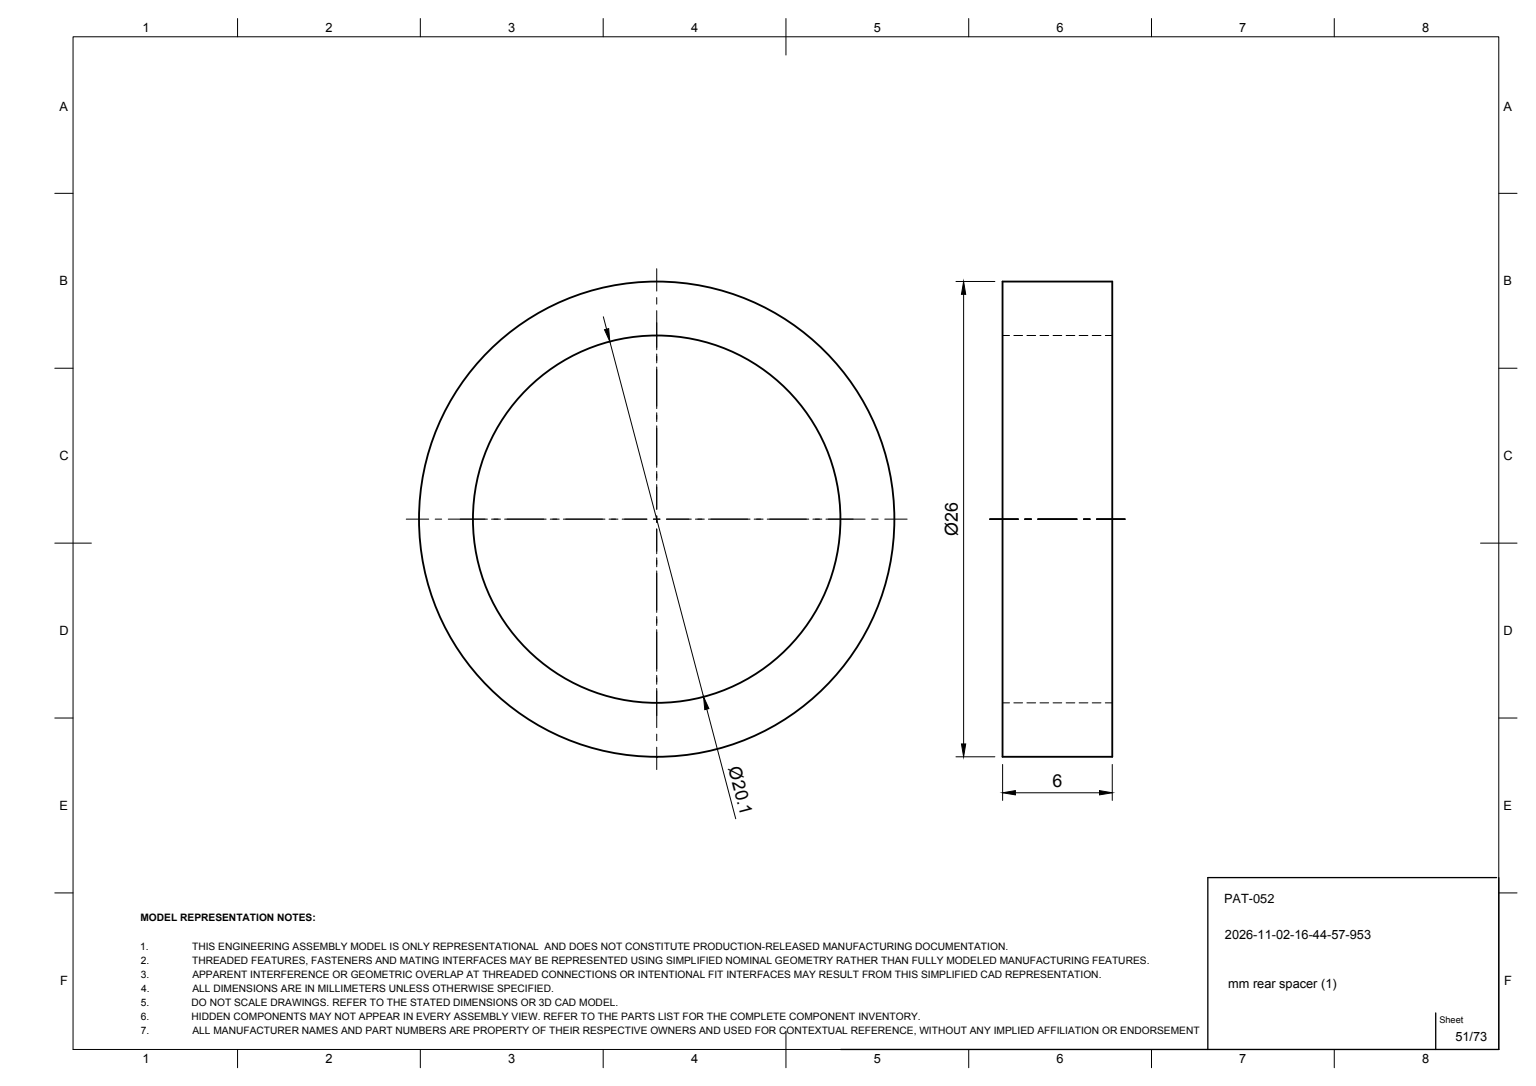
ISO-10303-21;
HEADER;
/* Generated by software containing ST-Developer
 * from STEP Tools, Inc. (www.steptools.com) 
 */

FILE_DESCRIPTION(
/* description */ ('Hand-crank gear train demonstrator'),
/* implementation_level */ '2;1');

FILE_NAME(
/* name */ 'mm rear spacer (1).step',
/* time_stamp */ '2026-10-28T03:22:13-07:00',
/* author */ (''),
/* organization */ (''),
/* preprocessor_version */ 'ST-DEVELOPER v20.2',
/* originating_system */ 'Autodesk Translation Framework v15.17.0.0',
/* authorisation */ '');

FILE_SCHEMA (('AUTOMOTIVE_DESIGN { 1 0 10303 214 3 1 1 }'));
ENDSEC;

DATA;
#10=MECHANICAL_DESIGN_GEOMETRIC_PRESENTATION_REPRESENTATION('',(#1245),#62758);
#1102=SHAPE_REPRESENTATION_RELATIONSHIP('SRR','None',#63078,#1166);
#1166=ADVANCED_BREP_SHAPE_REPRESENTATION('',(#1320),#62732);
#1245=STYLED_ITEM('',(#63476),#1320);
#1320=MANIFOLD_SOLID_BREP('Body1',#16429);
#1578=FACE_BOUND('',#3825,.T.);
#1579=FACE_BOUND('',#3827,.T.);
#1949=PLANE('',#18177);
#1950=PLANE('',#18178);
#2650=FACE_OUTER_BOUND('',#3822,.T.);
#2651=FACE_OUTER_BOUND('',#3823,.T.);
#2652=FACE_OUTER_BOUND('',#3824,.T.);
#2653=FACE_OUTER_BOUND('',#3826,.T.);
#3822=EDGE_LOOP('',(#13083,#13084,#13085,#13086));
#3823=EDGE_LOOP('',(#13087,#13088,#13089,#13090));
#3824=EDGE_LOOP('',(#13091));
#3825=EDGE_LOOP('',(#13092));
#3826=EDGE_LOOP('',(#13093));
#3827=EDGE_LOOP('',(#13094));
#4946=LINE('',#26469,#6078);
#4947=LINE('',#26475,#6079);
#6078=VECTOR('',#21521,1.005);
#6079=VECTOR('',#21528,1.3);
#6978=CIRCLE('',#18172,1.005);
#6979=CIRCLE('',#18173,1.005);
#6980=CIRCLE('',#18175,1.3);
#6981=CIRCLE('',#18176,1.3);
#7975=VERTEX_POINT('',#26466);
#7976=VERTEX_POINT('',#26468);
#7977=VERTEX_POINT('',#26472);
#7978=VERTEX_POINT('',#26474);
#9793=EDGE_CURVE('',#7975,#7975,#6978,.T.);
#9794=EDGE_CURVE('',#7975,#7976,#4946,.T.);
#9795=EDGE_CURVE('',#7976,#7976,#6979,.T.);
#9796=EDGE_CURVE('',#7977,#7977,#6980,.T.);
#9797=EDGE_CURVE('',#7977,#7978,#4947,.T.);
#9798=EDGE_CURVE('',#7978,#7978,#6981,.T.);
#13083=ORIENTED_EDGE('',*,*,#9793,.F.);
#13084=ORIENTED_EDGE('',*,*,#9794,.T.);
#13085=ORIENTED_EDGE('',*,*,#9795,.T.);
#13086=ORIENTED_EDGE('',*,*,#9794,.F.);
#13087=ORIENTED_EDGE('',*,*,#9796,.F.);
#13088=ORIENTED_EDGE('',*,*,#9797,.T.);
#13089=ORIENTED_EDGE('',*,*,#9798,.T.);
#13090=ORIENTED_EDGE('',*,*,#9797,.F.);
#13091=ORIENTED_EDGE('',*,*,#9796,.T.);
#13092=ORIENTED_EDGE('',*,*,#9793,.T.);
#13093=ORIENTED_EDGE('',*,*,#9798,.F.);
#13094=ORIENTED_EDGE('',*,*,#9795,.F.);
#15324=CYLINDRICAL_SURFACE('',#18171,1.005);
#15325=CYLINDRICAL_SURFACE('',#18174,1.3);
#15960=ADVANCED_FACE('',(#2650),#15324,.F.);
#15961=ADVANCED_FACE('',(#2651),#15325,.T.);
#15962=ADVANCED_FACE('',(#2652,#1578),#1949,.T.);
#15963=ADVANCED_FACE('',(#2653,#1579),#1950,.F.);
#16429=CLOSED_SHELL('',(#15960,#15961,#15962,#15963));
#18170=AXIS2_PLACEMENT_3D('',#26464,#21515,#21516);
#18171=AXIS2_PLACEMENT_3D('',#26465,#21517,#21518);
#18172=AXIS2_PLACEMENT_3D('',#26467,#21519,#21520);
#18173=AXIS2_PLACEMENT_3D('',#26470,#21522,#21523);
#18174=AXIS2_PLACEMENT_3D('',#26471,#21524,#21525);
#18175=AXIS2_PLACEMENT_3D('',#26473,#21526,#21527);
#18176=AXIS2_PLACEMENT_3D('',#26476,#21529,#21530);
#18177=AXIS2_PLACEMENT_3D('',#26477,#21531,#21532);
#18178=AXIS2_PLACEMENT_3D('',#26478,#21533,#21534);
#21515=DIRECTION('axis',(0.,0.,1.));
#21516=DIRECTION('refdir',(1.,0.,0.));
#21517=DIRECTION('center_axis',(0.,1.,0.));
#21518=DIRECTION('ref_axis',(1.,0.,0.));
#21519=DIRECTION('center_axis',(0.,-1.,0.));
#21520=DIRECTION('ref_axis',(1.,0.,0.));
#21521=DIRECTION('',(0.,-1.,0.));
#21522=DIRECTION('center_axis',(0.,-1.,0.));
#21523=DIRECTION('ref_axis',(1.,0.,0.));
#21524=DIRECTION('center_axis',(0.,1.,0.));
#21525=DIRECTION('ref_axis',(1.,0.,0.));
#21526=DIRECTION('center_axis',(0.,1.,0.));
#21527=DIRECTION('ref_axis',(1.,0.,0.));
#21528=DIRECTION('',(0.,-1.,0.));
#21529=DIRECTION('center_axis',(0.,1.,0.));
#21530=DIRECTION('ref_axis',(1.,0.,0.));
#21531=DIRECTION('center_axis',(0.,1.,0.));
#21532=DIRECTION('ref_axis',(1.,0.,0.));
#21533=DIRECTION('center_axis',(0.,1.,0.));
#21534=DIRECTION('ref_axis',(1.,0.,0.));
#26464=CARTESIAN_POINT('',(0.,0.,0.));
#26465=CARTESIAN_POINT('Origin',(6.,-2.8,9.));
#26466=CARTESIAN_POINT('',(4.995,-2.2,9.));
#26467=CARTESIAN_POINT('Origin',(6.,-2.2,9.));
#26468=CARTESIAN_POINT('',(4.995,-2.8,9.));
#26469=CARTESIAN_POINT('',(4.995,-2.8,9.));
#26470=CARTESIAN_POINT('Origin',(6.,-2.8,9.));
#26471=CARTESIAN_POINT('Origin',(6.,-2.8,9.));
#26472=CARTESIAN_POINT('',(4.7,-2.2,9.));
#26473=CARTESIAN_POINT('Origin',(6.,-2.2,9.));
#26474=CARTESIAN_POINT('',(4.7,-2.8,9.));
#26475=CARTESIAN_POINT('',(4.7,-2.8,9.));
#26476=CARTESIAN_POINT('Origin',(6.,-2.8,9.));
#26477=CARTESIAN_POINT('Origin',(6.,-2.2,9.));
#26478=CARTESIAN_POINT('Origin',(6.,-2.8,9.));
#62658=UNCERTAINTY_MEASURE_WITH_UNIT(LENGTH_MEASURE(0.001),#62759,
'DISTANCE_ACCURACY_VALUE',
'Maximum model space distance between geometric entities at asserted c
onnectivities');
#62684=UNCERTAINTY_MEASURE_WITH_UNIT(LENGTH_MEASURE(0.001),#62759,
'DISTANCE_ACCURACY_VALUE',
'Maximum model space distance between geometric entities at asserted c
onnectivities');
#62732=(
GEOMETRIC_REPRESENTATION_CONTEXT(3)
GLOBAL_UNCERTAINTY_ASSIGNED_CONTEXT((#62658))
GLOBAL_UNIT_ASSIGNED_CONTEXT((#62759,#62761,#62762))
REPRESENTATION_CONTEXT('','3D')
);
#62758=(
GEOMETRIC_REPRESENTATION_CONTEXT(3)
GLOBAL_UNCERTAINTY_ASSIGNED_CONTEXT((#62684))
GLOBAL_UNIT_ASSIGNED_CONTEXT((#62759,#62761,#62762))
REPRESENTATION_CONTEXT('','3D')
);
#62759=(
LENGTH_UNIT()
NAMED_UNIT(*)
SI_UNIT(.CENTI.,.METRE.)
);
#62761=(
NAMED_UNIT(*)
PLANE_ANGLE_UNIT()
SI_UNIT($,.RADIAN.)
);
#62762=(
NAMED_UNIT(*)
SI_UNIT($,.STERADIAN.)
SOLID_ANGLE_UNIT()
);
#62810=SHAPE_DEFINITION_REPRESENTATION(#62893,#63078);
#62893=PRODUCT_DEFINITION_SHAPE('',$,#63152);
#63078=SHAPE_REPRESENTATION('',(#18170),#62732);
#63104=PRODUCT_DEFINITION_CONTEXT('part definition',#63325,'design');
#63152=PRODUCT_DEFINITION('mm rear spacer (1)','mm rear spacer (1)',#63225,
#63104);
#63225=PRODUCT_DEFINITION_FORMATION('',$,#63374);
#63325=APPLICATION_CONTEXT(
'Core Data for Automotive Mechanical Design Process');
#63326=PRODUCT_CONTEXT('part definition',#63325,'mechanical');
#63374=PRODUCT('mm rear spacer (1)','mm rear spacer (1)','mm rear spacer (1)',
(#63326));
#63470=COLOUR_RGB('Off White',0.89,0.88,0.83);
#63471=FILL_AREA_STYLE_COLOUR('',#63470);
#63472=FILL_AREA_STYLE('',(#63471));
#63473=SURFACE_STYLE_FILL_AREA(#63472);
#63474=SURFACE_SIDE_STYLE('',(#63473));
#63475=SURFACE_STYLE_USAGE(.BOTH.,#63474);
#63476=PRESENTATION_STYLE_ASSIGNMENT((#63475));
ENDSEC;
END-ISO-10303-21;
